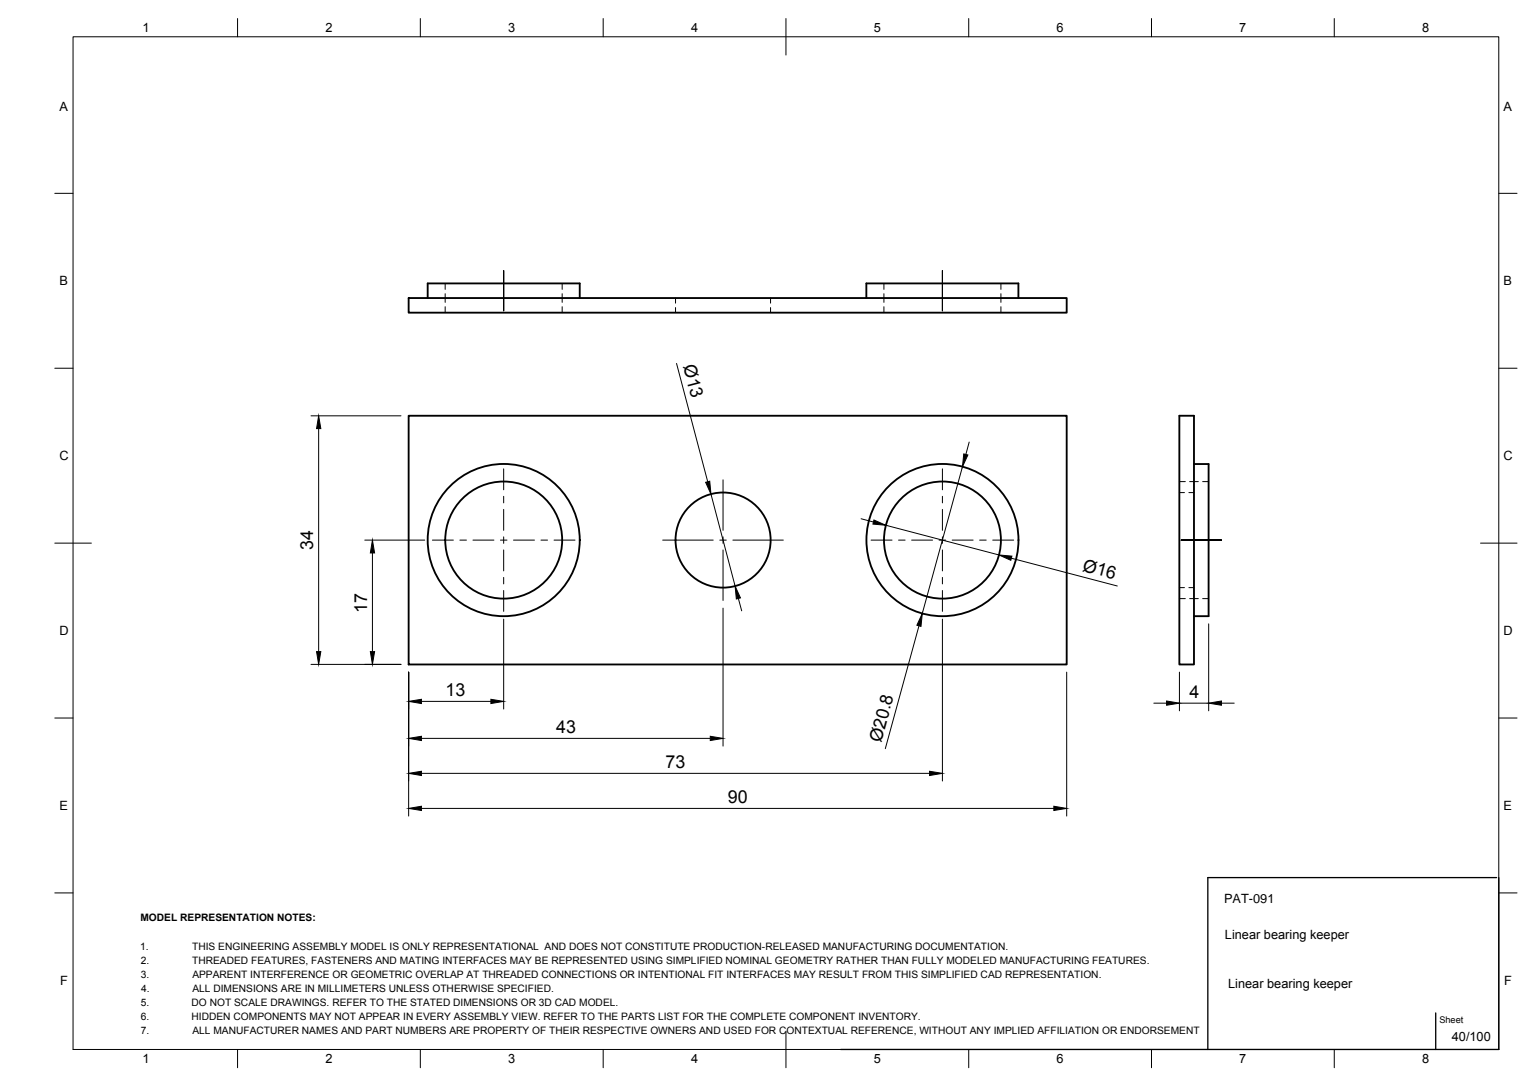
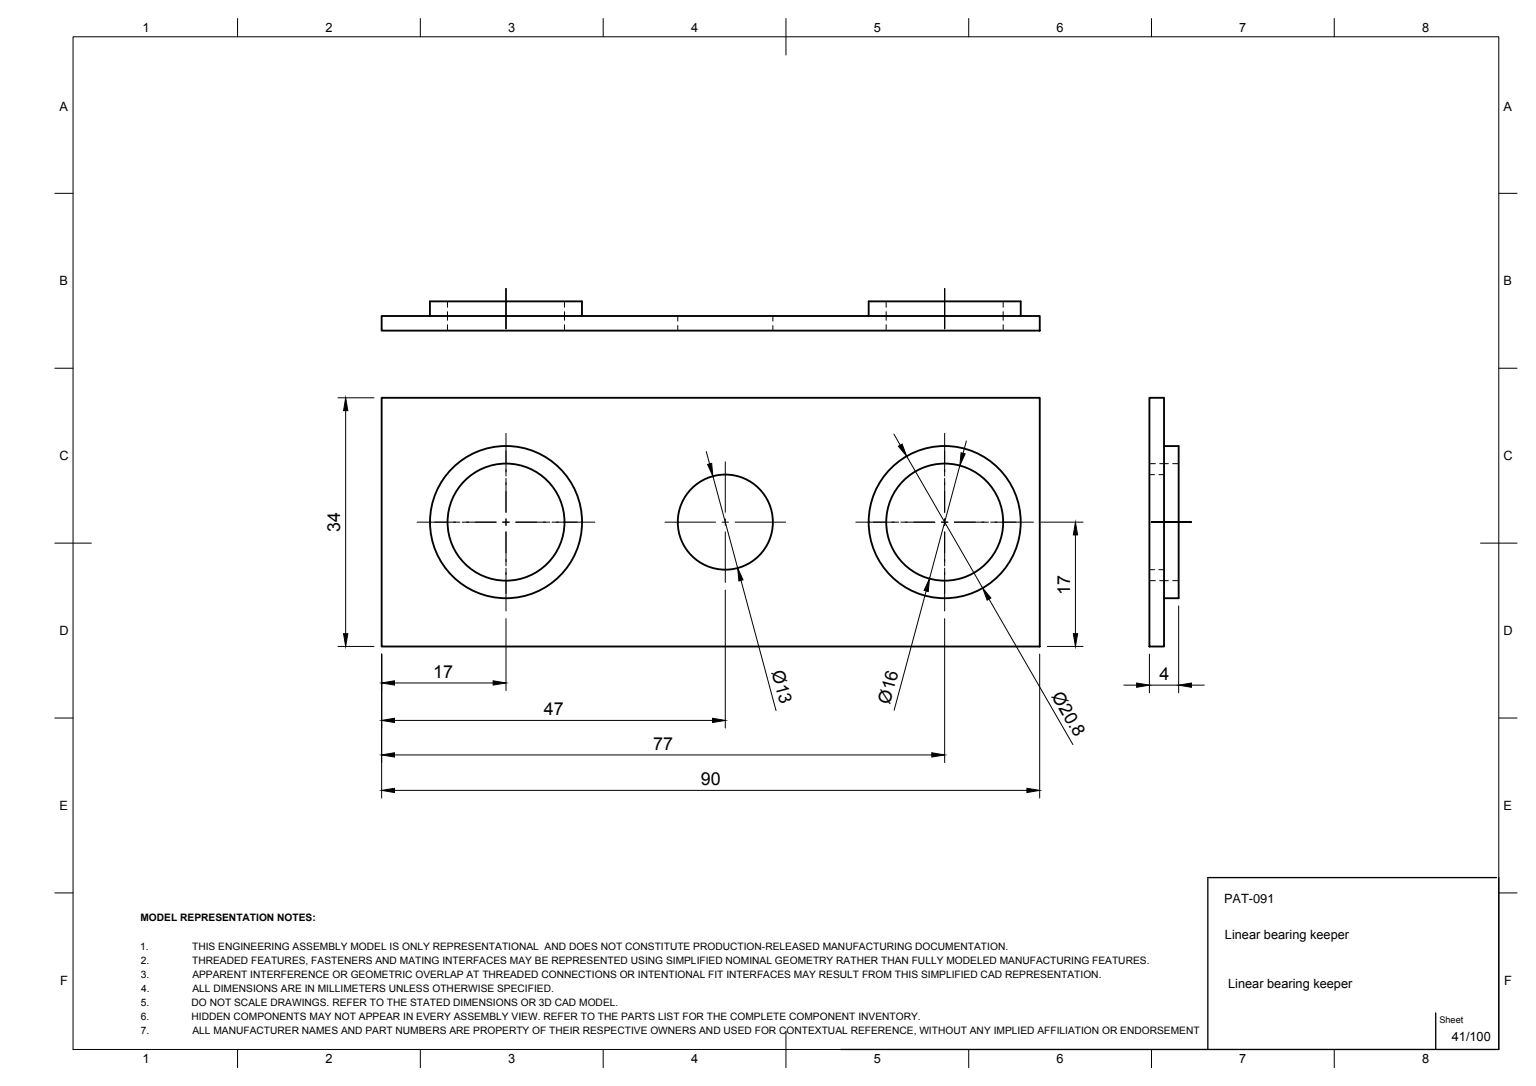
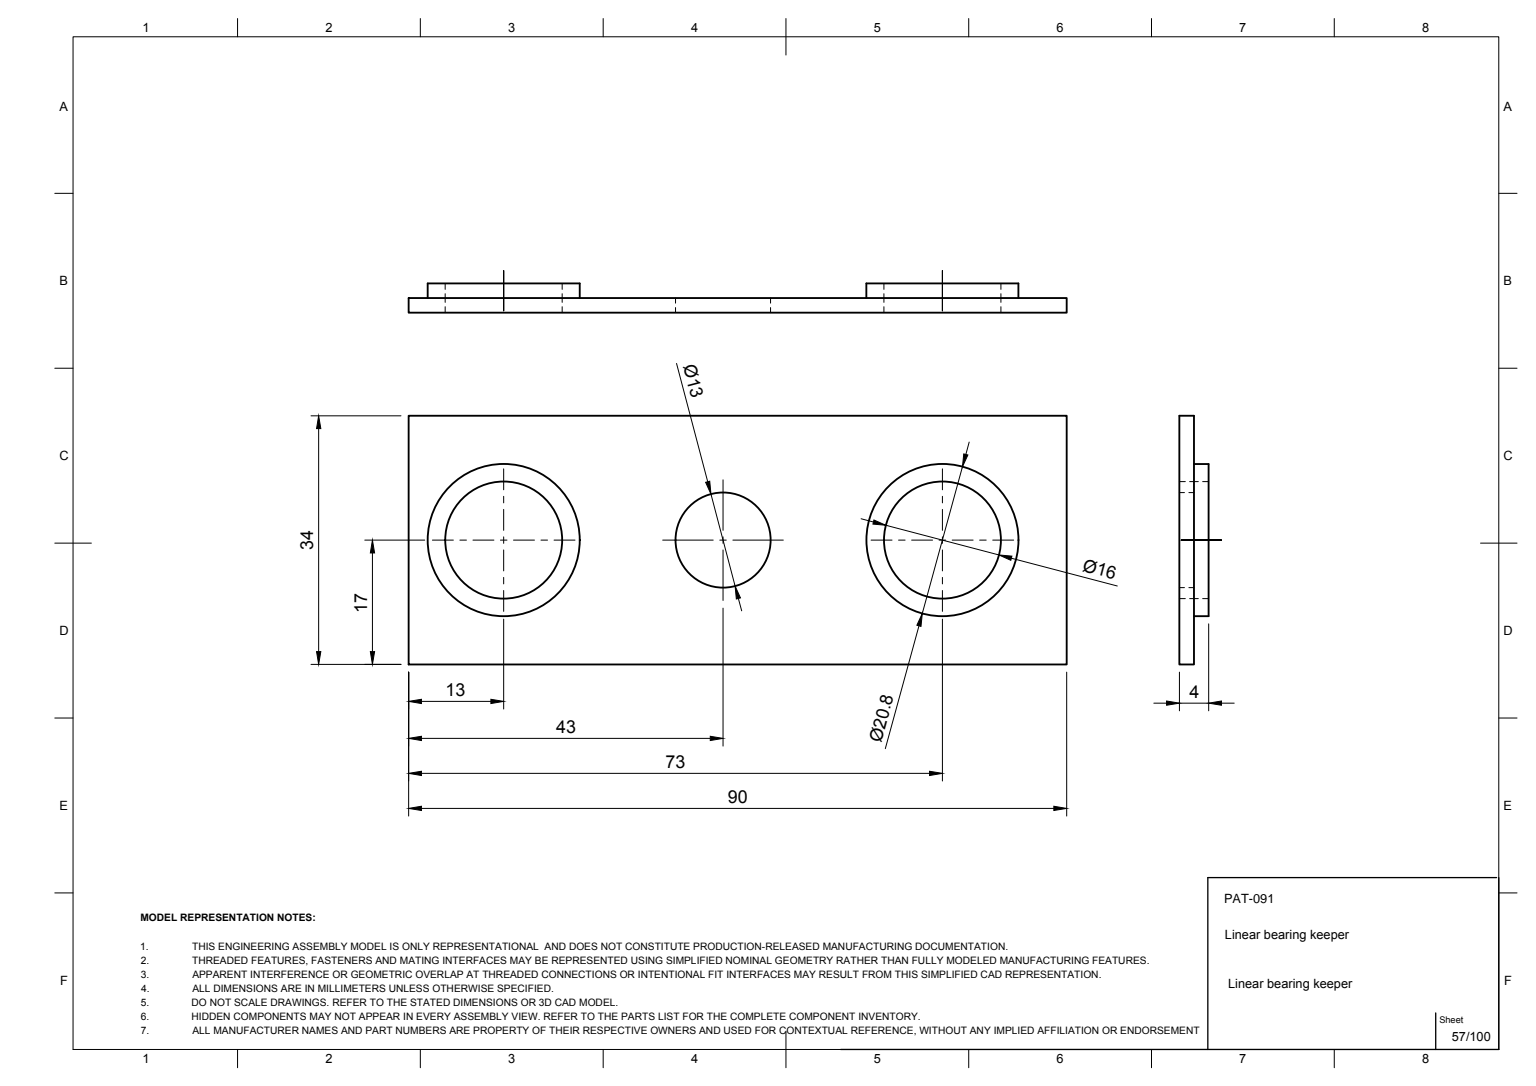
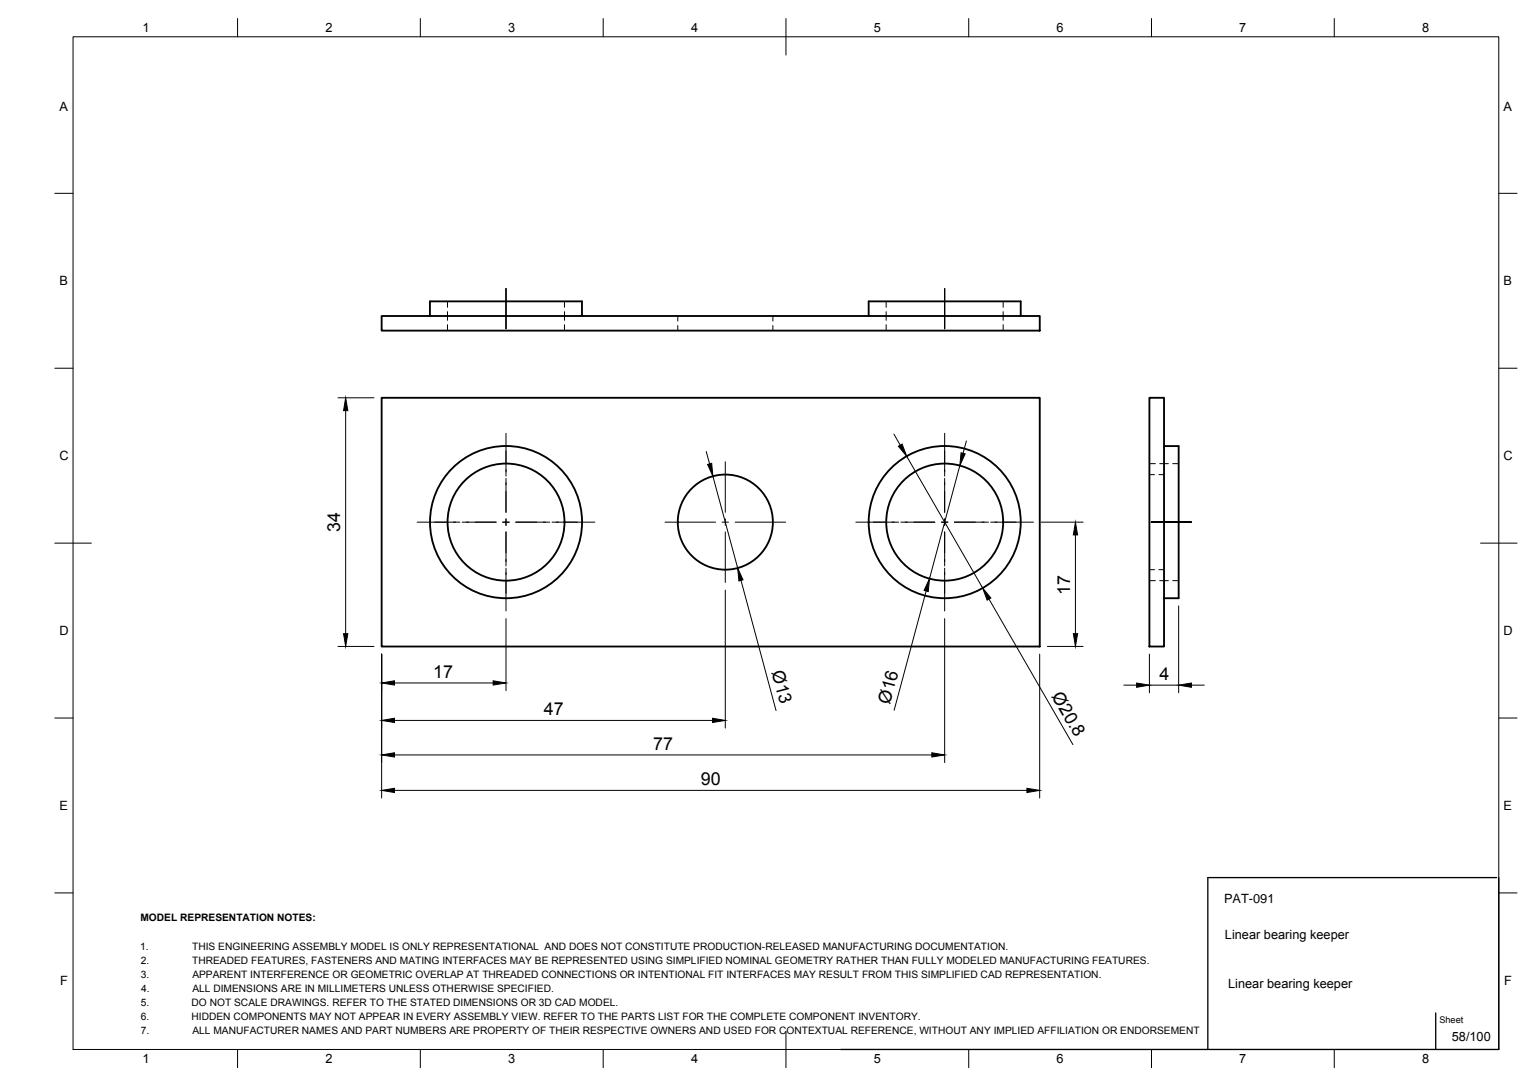
ISO-10303-21;
HEADER;
/* Generated by software containing ST-Developer
 * from STEP Tools, Inc. (www.steptools.com) 
 */

FILE_DESCRIPTION(
/* description */ ('PAT-091'),
/* implementation_level */ '2;1');

FILE_NAME(
/* name */ 'Linear bearing keeper.step',
/* time_stamp */ '2026-10-27T15:34:44-07:00',
/* author */ (''),
/* organization */ (''),
/* preprocessor_version */ 'ST-DEVELOPER v20.2',
/* originating_system */ 'Autodesk Translation Framework v15.17.0.0',
/* authorisation */ '');

FILE_SCHEMA (('AUTOMOTIVE_DESIGN { 1 0 10303 214 3 1 1 }'));
ENDSEC;

DATA;
#10=MECHANICAL_DESIGN_GEOMETRIC_PRESENTATION_REPRESENTATION('',(#1003),#25100);
#783=SHAPE_REPRESENTATION_RELATIONSHIP('SRR','None',#25546,#893);
#893=ADVANCED_BREP_SHAPE_REPRESENTATION('',(#1125),#25016);
#1003=STYLED_ITEM('',(#26191),#1125);
#1125=MANIFOLD_SOLID_BREP('Body1',#13282);
#1398=FACE_BOUND('',#3335,.T.);
#1399=FACE_BOUND('',#3338,.T.);
#1400=FACE_BOUND('',#3347,.T.);
#1401=FACE_BOUND('',#3348,.T.);
#1402=FACE_BOUND('',#3349,.T.);
#1403=FACE_BOUND('',#3351,.T.);
#1404=FACE_BOUND('',#3352,.T.);
#1405=FACE_BOUND('',#3353,.T.);
#1783=PLANE('',#15139);
#1784=PLANE('',#15144);
#1785=PLANE('',#15153);
#1786=PLANE('',#15154);
#1787=PLANE('',#15155);
#1788=PLANE('',#15156);
#1789=PLANE('',#15157);
#1790=PLANE('',#15158);
#2332=FACE_OUTER_BOUND('',#3333,.T.);
#2333=FACE_OUTER_BOUND('',#3334,.T.);
#2334=FACE_OUTER_BOUND('',#3336,.T.);
#2335=FACE_OUTER_BOUND('',#3337,.T.);
#2336=FACE_OUTER_BOUND('',#3339,.T.);
#2337=FACE_OUTER_BOUND('',#3340,.T.);
#2338=FACE_OUTER_BOUND('',#3341,.T.);
#2339=FACE_OUTER_BOUND('',#3342,.T.);
#2340=FACE_OUTER_BOUND('',#3343,.T.);
#2341=FACE_OUTER_BOUND('',#3344,.T.);
#2342=FACE_OUTER_BOUND('',#3345,.T.);
#2343=FACE_OUTER_BOUND('',#3346,.T.);
#2344=FACE_OUTER_BOUND('',#3350,.T.);
#3333=EDGE_LOOP('',(#10098,#10099,#10100,#10101));
#3334=EDGE_LOOP('',(#10102));
#3335=EDGE_LOOP('',(#10103));
#3336=EDGE_LOOP('',(#10104,#10105,#10106,#10107));
#3337=EDGE_LOOP('',(#10108));
#3338=EDGE_LOOP('',(#10109));
#3339=EDGE_LOOP('',(#10110,#10111,#10112,#10113));
#3340=EDGE_LOOP('',(#10114,#10115,#10116,#10117));
#3341=EDGE_LOOP('',(#10118,#10119,#10120,#10121));
#3342=EDGE_LOOP('',(#10122,#10123,#10124,#10125));
#3343=EDGE_LOOP('',(#10126,#10127,#10128,#10129));
#3344=EDGE_LOOP('',(#10130,#10131,#10132,#10133));
#3345=EDGE_LOOP('',(#10134,#10135,#10136,#10137));
#3346=EDGE_LOOP('',(#10138,#10139,#10140,#10141));
#3347=EDGE_LOOP('',(#10142));
#3348=EDGE_LOOP('',(#10143));
#3349=EDGE_LOOP('',(#10144));
#3350=EDGE_LOOP('',(#10145,#10146,#10147,#10148));
#3351=EDGE_LOOP('',(#10149));
#3352=EDGE_LOOP('',(#10150));
#3353=EDGE_LOOP('',(#10151));
#4442=LINE('',#22220,#5182);
#4443=LINE('',#22229,#5183);
#4444=LINE('',#22238,#5184);
#4445=LINE('',#22243,#5185);
#4446=LINE('',#22247,#5186);
#4447=LINE('',#22251,#5187);
#4448=LINE('',#22253,#5188);
#4449=LINE('',#22255,#5189);
#4450=LINE('',#22256,#5190);
#4451=LINE('',#22259,#5191);
#4452=LINE('',#22261,#5192);
#4453=LINE('',#22262,#5193);
#4454=LINE('',#22265,#5194);
#4455=LINE('',#22267,#5195);
#4456=LINE('',#22268,#5196);
#4457=LINE('',#22270,#5197);
#4458=LINE('',#22271,#5198);
#5182=VECTOR('',#17892,1.04);
#5183=VECTOR('',#17903,1.04);
#5184=VECTOR('',#17914,0.65);
#5185=VECTOR('',#17921,0.8);
#5186=VECTOR('',#17926,0.8);
#5187=VECTOR('',#17929,1.);
#5188=VECTOR('',#17930,1.);
#5189=VECTOR('',#17931,1.);
#5190=VECTOR('',#17932,1.);
#5191=VECTOR('',#17935,1.);
#5192=VECTOR('',#17936,1.);
#5193=VECTOR('',#17937,1.);
#5194=VECTOR('',#17940,1.);
#5195=VECTOR('',#17941,1.);
#5196=VECTOR('',#17942,1.);
#5197=VECTOR('',#17945,1.);
#5198=VECTOR('',#17946,1.);
#5849=CIRCLE('',#15137,1.04);
#5850=CIRCLE('',#15138,1.04);
#5851=CIRCLE('',#15140,0.8);
#5852=CIRCLE('',#15142,1.04);
#5853=CIRCLE('',#15143,1.04);
#5854=CIRCLE('',#15145,0.8);
#5855=CIRCLE('',#15147,0.65);
#5856=CIRCLE('',#15148,0.65);
#5857=CIRCLE('',#15150,0.8);
#5858=CIRCLE('',#15152,0.8);
#6756=VERTEX_POINT('',#22217);
#6757=VERTEX_POINT('',#22219);
#6758=VERTEX_POINT('',#22223);
#6759=VERTEX_POINT('',#22226);
#6760=VERTEX_POINT('',#22228);
#6761=VERTEX_POINT('',#22232);
#6762=VERTEX_POINT('',#22235);
#6763=VERTEX_POINT('',#22237);
#6764=VERTEX_POINT('',#22241);
#6765=VERTEX_POINT('',#22245);
#6766=VERTEX_POINT('',#22249);
#6767=VERTEX_POINT('',#22250);
#6768=VERTEX_POINT('',#22252);
#6769=VERTEX_POINT('',#22254);
#6770=VERTEX_POINT('',#22258);
#6771=VERTEX_POINT('',#22260);
#6772=VERTEX_POINT('',#22264);
#6773=VERTEX_POINT('',#22266);
#7984=EDGE_CURVE('',#6756,#6756,#5849,.T.);
#7985=EDGE_CURVE('',#6756,#6757,#4442,.T.);
#7986=EDGE_CURVE('',#6757,#6757,#5850,.T.);
#7987=EDGE_CURVE('',#6758,#6758,#5851,.T.);
#7988=EDGE_CURVE('',#6759,#6759,#5852,.T.);
#7989=EDGE_CURVE('',#6759,#6760,#4443,.T.);
#7990=EDGE_CURVE('',#6760,#6760,#5853,.T.);
#7991=EDGE_CURVE('',#6761,#6761,#5854,.T.);
#7992=EDGE_CURVE('',#6762,#6762,#5855,.T.);
#7993=EDGE_CURVE('',#6762,#6763,#4444,.T.);
#7994=EDGE_CURVE('',#6763,#6763,#5856,.T.);
#7995=EDGE_CURVE('',#6764,#6764,#5857,.T.);
#7996=EDGE_CURVE('',#6764,#6761,#4445,.T.);
#7997=EDGE_CURVE('',#6765,#6765,#5858,.T.);
#7998=EDGE_CURVE('',#6765,#6758,#4446,.T.);
#7999=EDGE_CURVE('',#6766,#6767,#4447,.T.);
#8000=EDGE_CURVE('',#6767,#6768,#4448,.T.);
#8001=EDGE_CURVE('',#6769,#6768,#4449,.T.);
#8002=EDGE_CURVE('',#6766,#6769,#4450,.T.);
#8003=EDGE_CURVE('',#6770,#6766,#4451,.T.);
#8004=EDGE_CURVE('',#6771,#6769,#4452,.T.);
#8005=EDGE_CURVE('',#6770,#6771,#4453,.T.);
#8006=EDGE_CURVE('',#6772,#6770,#4454,.T.);
#8007=EDGE_CURVE('',#6773,#6771,#4455,.T.);
#8008=EDGE_CURVE('',#6772,#6773,#4456,.T.);
#8009=EDGE_CURVE('',#6767,#6772,#4457,.T.);
#8010=EDGE_CURVE('',#6768,#6773,#4458,.T.);
#10098=ORIENTED_EDGE('',*,*,#7984,.F.);
#10099=ORIENTED_EDGE('',*,*,#7985,.T.);
#10100=ORIENTED_EDGE('',*,*,#7986,.F.);
#10101=ORIENTED_EDGE('',*,*,#7985,.F.);
#10102=ORIENTED_EDGE('',*,*,#7984,.T.);
#10103=ORIENTED_EDGE('',*,*,#7987,.T.);
#10104=ORIENTED_EDGE('',*,*,#7988,.F.);
#10105=ORIENTED_EDGE('',*,*,#7989,.T.);
#10106=ORIENTED_EDGE('',*,*,#7990,.F.);
#10107=ORIENTED_EDGE('',*,*,#7989,.F.);
#10108=ORIENTED_EDGE('',*,*,#7988,.T.);
#10109=ORIENTED_EDGE('',*,*,#7991,.T.);
#10110=ORIENTED_EDGE('',*,*,#7992,.F.);
#10111=ORIENTED_EDGE('',*,*,#7993,.T.);
#10112=ORIENTED_EDGE('',*,*,#7994,.F.);
#10113=ORIENTED_EDGE('',*,*,#7993,.F.);
#10114=ORIENTED_EDGE('',*,*,#7995,.F.);
#10115=ORIENTED_EDGE('',*,*,#7996,.T.);
#10116=ORIENTED_EDGE('',*,*,#7991,.F.);
#10117=ORIENTED_EDGE('',*,*,#7996,.F.);
#10118=ORIENTED_EDGE('',*,*,#7997,.F.);
#10119=ORIENTED_EDGE('',*,*,#7998,.T.);
#10120=ORIENTED_EDGE('',*,*,#7987,.F.);
#10121=ORIENTED_EDGE('',*,*,#7998,.F.);
#10122=ORIENTED_EDGE('',*,*,#7999,.T.);
#10123=ORIENTED_EDGE('',*,*,#8000,.T.);
#10124=ORIENTED_EDGE('',*,*,#8001,.F.);
#10125=ORIENTED_EDGE('',*,*,#8002,.F.);
#10126=ORIENTED_EDGE('',*,*,#8003,.T.);
#10127=ORIENTED_EDGE('',*,*,#8002,.T.);
#10128=ORIENTED_EDGE('',*,*,#8004,.F.);
#10129=ORIENTED_EDGE('',*,*,#8005,.F.);
#10130=ORIENTED_EDGE('',*,*,#8006,.T.);
#10131=ORIENTED_EDGE('',*,*,#8005,.T.);
#10132=ORIENTED_EDGE('',*,*,#8007,.F.);
#10133=ORIENTED_EDGE('',*,*,#8008,.F.);
#10134=ORIENTED_EDGE('',*,*,#8009,.T.);
#10135=ORIENTED_EDGE('',*,*,#8008,.T.);
#10136=ORIENTED_EDGE('',*,*,#8010,.F.);
#10137=ORIENTED_EDGE('',*,*,#8000,.F.);
#10138=ORIENTED_EDGE('',*,*,#8010,.T.);
#10139=ORIENTED_EDGE('',*,*,#8007,.T.);
#10140=ORIENTED_EDGE('',*,*,#8004,.T.);
#10141=ORIENTED_EDGE('',*,*,#8001,.T.);
#10142=ORIENTED_EDGE('',*,*,#7986,.T.);
#10143=ORIENTED_EDGE('',*,*,#7990,.T.);
#10144=ORIENTED_EDGE('',*,*,#7994,.T.);
#10145=ORIENTED_EDGE('',*,*,#8009,.F.);
#10146=ORIENTED_EDGE('',*,*,#7999,.F.);
#10147=ORIENTED_EDGE('',*,*,#8003,.F.);
#10148=ORIENTED_EDGE('',*,*,#8006,.F.);
#10149=ORIENTED_EDGE('',*,*,#7992,.T.);
#10150=ORIENTED_EDGE('',*,*,#7995,.T.);
#10151=ORIENTED_EDGE('',*,*,#7997,.T.);
#12193=CYLINDRICAL_SURFACE('',#15136,1.04);
#12194=CYLINDRICAL_SURFACE('',#15141,1.04);
#12195=CYLINDRICAL_SURFACE('',#15146,0.65);
#12196=CYLINDRICAL_SURFACE('',#15149,0.8);
#12197=CYLINDRICAL_SURFACE('',#15151,0.8);
#12699=ADVANCED_FACE('',(#2332),#12193,.T.);
#12700=ADVANCED_FACE('',(#2333,#1398),#1783,.T.);
#12701=ADVANCED_FACE('',(#2334),#12194,.T.);
#12702=ADVANCED_FACE('',(#2335,#1399),#1784,.T.);
#12703=ADVANCED_FACE('',(#2336),#12195,.F.);
#12704=ADVANCED_FACE('',(#2337),#12196,.F.);
#12705=ADVANCED_FACE('',(#2338),#12197,.F.);
#12706=ADVANCED_FACE('',(#2339),#1785,.T.);
#12707=ADVANCED_FACE('',(#2340),#1786,.T.);
#12708=ADVANCED_FACE('',(#2341),#1787,.T.);
#12709=ADVANCED_FACE('',(#2342),#1788,.T.);
#12710=ADVANCED_FACE('',(#2343,#1400,#1401,#1402),#1789,.T.);
#12711=ADVANCED_FACE('',(#2344,#1403,#1404,#1405),#1790,.F.);
#13282=CLOSED_SHELL('',(#12699,#12700,#12701,#12702,#12703,#12704,#12705,
#12706,#12707,#12708,#12709,#12710,#12711));
#15135=AXIS2_PLACEMENT_3D('',#22215,#17886,#17887);
#15136=AXIS2_PLACEMENT_3D('',#22216,#17888,#17889);
#15137=AXIS2_PLACEMENT_3D('',#22218,#17890,#17891);
#15138=AXIS2_PLACEMENT_3D('',#22221,#17893,#17894);
#15139=AXIS2_PLACEMENT_3D('',#22222,#17895,#17896);
#15140=AXIS2_PLACEMENT_3D('',#22224,#17897,#17898);
#15141=AXIS2_PLACEMENT_3D('',#22225,#17899,#17900);
#15142=AXIS2_PLACEMENT_3D('',#22227,#17901,#17902);
#15143=AXIS2_PLACEMENT_3D('',#22230,#17904,#17905);
#15144=AXIS2_PLACEMENT_3D('',#22231,#17906,#17907);
#15145=AXIS2_PLACEMENT_3D('',#22233,#17908,#17909);
#15146=AXIS2_PLACEMENT_3D('',#22234,#17910,#17911);
#15147=AXIS2_PLACEMENT_3D('',#22236,#17912,#17913);
#15148=AXIS2_PLACEMENT_3D('',#22239,#17915,#17916);
#15149=AXIS2_PLACEMENT_3D('',#22240,#17917,#17918);
#15150=AXIS2_PLACEMENT_3D('',#22242,#17919,#17920);
#15151=AXIS2_PLACEMENT_3D('',#22244,#17922,#17923);
#15152=AXIS2_PLACEMENT_3D('',#22246,#17924,#17925);
#15153=AXIS2_PLACEMENT_3D('',#22248,#17927,#17928);
#15154=AXIS2_PLACEMENT_3D('',#22257,#17933,#17934);
#15155=AXIS2_PLACEMENT_3D('',#22263,#17938,#17939);
#15156=AXIS2_PLACEMENT_3D('',#22269,#17943,#17944);
#15157=AXIS2_PLACEMENT_3D('',#22272,#17947,#17948);
#15158=AXIS2_PLACEMENT_3D('',#22273,#17949,#17950);
#17886=DIRECTION('axis',(0.,0.,1.));
#17887=DIRECTION('refdir',(1.,0.,0.));
#17888=DIRECTION('center_axis',(1.,0.,0.));
#17889=DIRECTION('ref_axis',(0.,0.,-1.));
#17890=DIRECTION('center_axis',(1.,0.,0.));
#17891=DIRECTION('ref_axis',(0.,0.,-1.));
#17892=DIRECTION('',(-1.,0.,0.));
#17893=DIRECTION('center_axis',(-1.,0.,0.));
#17894=DIRECTION('ref_axis',(0.,0.,-1.));
#17895=DIRECTION('center_axis',(1.,0.,0.));
#17896=DIRECTION('ref_axis',(0.,0.,-1.));
#17897=DIRECTION('center_axis',(-1.,0.,0.));
#17898=DIRECTION('ref_axis',(0.,0.,-1.));
#17899=DIRECTION('center_axis',(1.,0.,0.));
#17900=DIRECTION('ref_axis',(0.,0.,-1.));
#17901=DIRECTION('center_axis',(1.,0.,0.));
#17902=DIRECTION('ref_axis',(0.,0.,-1.));
#17903=DIRECTION('',(-1.,0.,0.));
#17904=DIRECTION('center_axis',(-1.,0.,0.));
#17905=DIRECTION('ref_axis',(0.,0.,-1.));
#17906=DIRECTION('center_axis',(1.,0.,0.));
#17907=DIRECTION('ref_axis',(0.,0.,-1.));
#17908=DIRECTION('center_axis',(-1.,0.,0.));
#17909=DIRECTION('ref_axis',(0.,0.,-1.));
#17910=DIRECTION('center_axis',(1.,0.,0.));
#17911=DIRECTION('ref_axis',(0.,0.,-1.));
#17912=DIRECTION('center_axis',(1.,0.,0.));
#17913=DIRECTION('ref_axis',(0.,0.,-1.));
#17914=DIRECTION('',(1.,0.,0.));
#17915=DIRECTION('center_axis',(-1.,0.,0.));
#17916=DIRECTION('ref_axis',(0.,0.,-1.));
#17917=DIRECTION('center_axis',(1.,0.,0.));
#17918=DIRECTION('ref_axis',(0.,0.,-1.));
#17919=DIRECTION('center_axis',(1.,0.,0.));
#17920=DIRECTION('ref_axis',(0.,0.,-1.));
#17921=DIRECTION('',(1.,0.,0.));
#17922=DIRECTION('center_axis',(1.,0.,0.));
#17923=DIRECTION('ref_axis',(0.,0.,-1.));
#17924=DIRECTION('center_axis',(1.,0.,0.));
#17925=DIRECTION('ref_axis',(0.,0.,-1.));
#17926=DIRECTION('',(1.,0.,0.));
#17927=DIRECTION('center_axis',(0.,0.,1.));
#17928=DIRECTION('ref_axis',(0.,-1.,0.));
#17929=DIRECTION('',(0.,-1.,0.));
#17930=DIRECTION('',(1.,0.,0.));
#17931=DIRECTION('',(0.,-1.,0.));
#17932=DIRECTION('',(1.,0.,0.));
#17933=DIRECTION('center_axis',(0.,1.,0.));
#17934=DIRECTION('ref_axis',(0.,0.,1.));
#17935=DIRECTION('',(0.,0.,1.));
#17936=DIRECTION('',(0.,0.,1.));
#17937=DIRECTION('',(1.,0.,0.));
#17938=DIRECTION('center_axis',(0.,0.,-1.));
#17939=DIRECTION('ref_axis',(0.,1.,0.));
#17940=DIRECTION('',(0.,1.,0.));
#17941=DIRECTION('',(0.,1.,0.));
#17942=DIRECTION('',(1.,0.,0.));
#17943=DIRECTION('center_axis',(0.,-1.,0.));
#17944=DIRECTION('ref_axis',(0.,0.,-1.));
#17945=DIRECTION('',(0.,0.,-1.));
#17946=DIRECTION('',(0.,0.,-1.));
#17947=DIRECTION('center_axis',(1.,0.,0.));
#17948=DIRECTION('ref_axis',(0.,0.,-1.));
#17949=DIRECTION('center_axis',(1.,0.,0.));
#17950=DIRECTION('ref_axis',(0.,0.,-1.));
#22215=CARTESIAN_POINT('',(0.,0.,0.));
#22216=CARTESIAN_POINT('Origin',(37.02983346,3.,6.));
#22217=CARTESIAN_POINT('',(37.22983346,3.,7.04));
#22218=CARTESIAN_POINT('Origin',(37.22983346,3.,6.));
#22219=CARTESIAN_POINT('',(37.02983346,3.,7.04));
#22220=CARTESIAN_POINT('',(37.02983346,3.,7.04));
#22221=CARTESIAN_POINT('Origin',(37.02983346,3.,6.));
#22222=CARTESIAN_POINT('Origin',(37.22983346,3.,6.));
#22223=CARTESIAN_POINT('',(37.22983346,3.,6.8));
#22224=CARTESIAN_POINT('Origin',(37.22983346,3.,6.));
#22225=CARTESIAN_POINT('Origin',(37.02983346,-3.,6.));
#22226=CARTESIAN_POINT('',(37.22983346,-3.,7.04));
#22227=CARTESIAN_POINT('Origin',(37.22983346,-3.,6.));
#22228=CARTESIAN_POINT('',(37.02983346,-3.,7.04));
#22229=CARTESIAN_POINT('',(37.02983346,-3.,7.04));
#22230=CARTESIAN_POINT('Origin',(37.02983346,-3.,6.));
#22231=CARTESIAN_POINT('Origin',(37.22983346,-3.,6.));
#22232=CARTESIAN_POINT('',(37.22983346,-3.,6.8));
#22233=CARTESIAN_POINT('Origin',(37.22983346,-3.,6.));
#22234=CARTESIAN_POINT('Origin',(36.72983346,0.,6.));
#22235=CARTESIAN_POINT('',(36.82983346,-7.9602041944578E-17,6.65));
#22236=CARTESIAN_POINT('Origin',(36.82983346,0.,6.));
#22237=CARTESIAN_POINT('',(37.02983346,7.9602041944578E-17,6.65));
#22238=CARTESIAN_POINT('',(36.72983346,-7.9602041944578E-17,6.65));
#22239=CARTESIAN_POINT('Origin',(37.02983346,0.,6.));
#22240=CARTESIAN_POINT('Origin',(36.72983346,-3.,6.));
#22241=CARTESIAN_POINT('',(36.82983346,-3.,6.8));
#22242=CARTESIAN_POINT('Origin',(36.82983346,-3.,6.));
#22243=CARTESIAN_POINT('',(36.72983346,-3.,6.8));
#22244=CARTESIAN_POINT('Origin',(36.72983346,3.,6.));
#22245=CARTESIAN_POINT('',(36.82983346,3.,6.8));
#22246=CARTESIAN_POINT('Origin',(36.82983346,3.,6.));
#22247=CARTESIAN_POINT('',(36.72983346,3.,6.8));
#22248=CARTESIAN_POINT('Origin',(36.82983346,4.7,7.7));
#22249=CARTESIAN_POINT('',(36.82983346,4.7,7.7));
#22250=CARTESIAN_POINT('',(36.82983346,-4.3,7.7));
#22251=CARTESIAN_POINT('',(36.82983346,4.7,7.7));
#22252=CARTESIAN_POINT('',(37.02983346,-4.3,7.7));
#22253=CARTESIAN_POINT('',(36.82983346,-4.3,7.7));
#22254=CARTESIAN_POINT('',(37.02983346,4.7,7.7));
#22255=CARTESIAN_POINT('',(37.02983346,4.7,7.7));
#22256=CARTESIAN_POINT('',(36.82983346,4.7,7.7));
#22257=CARTESIAN_POINT('Origin',(36.82983346,4.7,4.3));
#22258=CARTESIAN_POINT('',(36.82983346,4.7,4.3));
#22259=CARTESIAN_POINT('',(36.82983346,4.7,4.3));
#22260=CARTESIAN_POINT('',(37.02983346,4.7,4.3));
#22261=CARTESIAN_POINT('',(37.02983346,4.7,4.3));
#22262=CARTESIAN_POINT('',(36.82983346,4.7,4.3));
#22263=CARTESIAN_POINT('Origin',(36.82983346,-4.3,4.3));
#22264=CARTESIAN_POINT('',(36.82983346,-4.3,4.3));
#22265=CARTESIAN_POINT('',(36.82983346,-4.3,4.3));
#22266=CARTESIAN_POINT('',(37.02983346,-4.3,4.3));
#22267=CARTESIAN_POINT('',(37.02983346,-4.3,4.3));
#22268=CARTESIAN_POINT('',(36.82983346,-4.3,4.3));
#22269=CARTESIAN_POINT('Origin',(36.82983346,-4.3,7.7));
#22270=CARTESIAN_POINT('',(36.82983346,-4.3,7.7));
#22271=CARTESIAN_POINT('',(37.02983346,-4.3,7.7));
#22272=CARTESIAN_POINT('Origin',(37.02983346,0.2,6.));
#22273=CARTESIAN_POINT('Origin',(36.82983346,0.2,6.));
#24895=UNCERTAINTY_MEASURE_WITH_UNIT(LENGTH_MEASURE(0.001),#25101,
'DISTANCE_ACCURACY_VALUE',
'Maximum model space distance between geometric entities at asserted c
onnectivities');
#24979=UNCERTAINTY_MEASURE_WITH_UNIT(LENGTH_MEASURE(0.001),#25101,
'DISTANCE_ACCURACY_VALUE',
'Maximum model space distance between geometric entities at asserted c
onnectivities');
#25016=(
GEOMETRIC_REPRESENTATION_CONTEXT(3)
GLOBAL_UNCERTAINTY_ASSIGNED_CONTEXT((#24895))
GLOBAL_UNIT_ASSIGNED_CONTEXT((#25101,#25103,#25104))
REPRESENTATION_CONTEXT('','3D')
);
#25100=(
GEOMETRIC_REPRESENTATION_CONTEXT(3)
GLOBAL_UNCERTAINTY_ASSIGNED_CONTEXT((#24979))
GLOBAL_UNIT_ASSIGNED_CONTEXT((#25101,#25103,#25104))
REPRESENTATION_CONTEXT('','3D')
);
#25101=(
LENGTH_UNIT()
NAMED_UNIT(*)
SI_UNIT(.CENTI.,.METRE.)
);
#25103=(
NAMED_UNIT(*)
PLANE_ANGLE_UNIT()
SI_UNIT($,.RADIAN.)
);
#25104=(
NAMED_UNIT(*)
SI_UNIT($,.STERADIAN.)
SOLID_ANGLE_UNIT()
);
#25141=SHAPE_DEFINITION_REPRESENTATION(#25261,#25546);
#25261=PRODUCT_DEFINITION_SHAPE('',$,#25667);
#25546=SHAPE_REPRESENTATION('',(#15135),#25016);
#25630=PRODUCT_DEFINITION_CONTEXT('part definition',#25992,'design');
#25667=PRODUCT_DEFINITION('Linear bearing keeper',
'Linear bearing keeper',#25787,#25630);
#25787=PRODUCT_DEFINITION_FORMATION('',$,#26030);
#25992=APPLICATION_CONTEXT(
'Core Data for Automotive Mechanical Design Process');
#25993=PRODUCT_CONTEXT('part definition',#25992,'mechanical');
#26030=PRODUCT('Linear bearing keeper','Linear bearing keeper',
'Linear bearing keeper',(#25993));
#26185=COLOUR_RGB('Grey',0.48,0.52,0.57);
#26186=FILL_AREA_STYLE_COLOUR('',#26185);
#26187=FILL_AREA_STYLE('',(#26186));
#26188=SURFACE_STYLE_FILL_AREA(#26187);
#26189=SURFACE_SIDE_STYLE('',(#26188));
#26190=SURFACE_STYLE_USAGE(.BOTH.,#26189);
#26191=PRESENTATION_STYLE_ASSIGNMENT((#26190));
ENDSEC;
END-ISO-10303-21;
